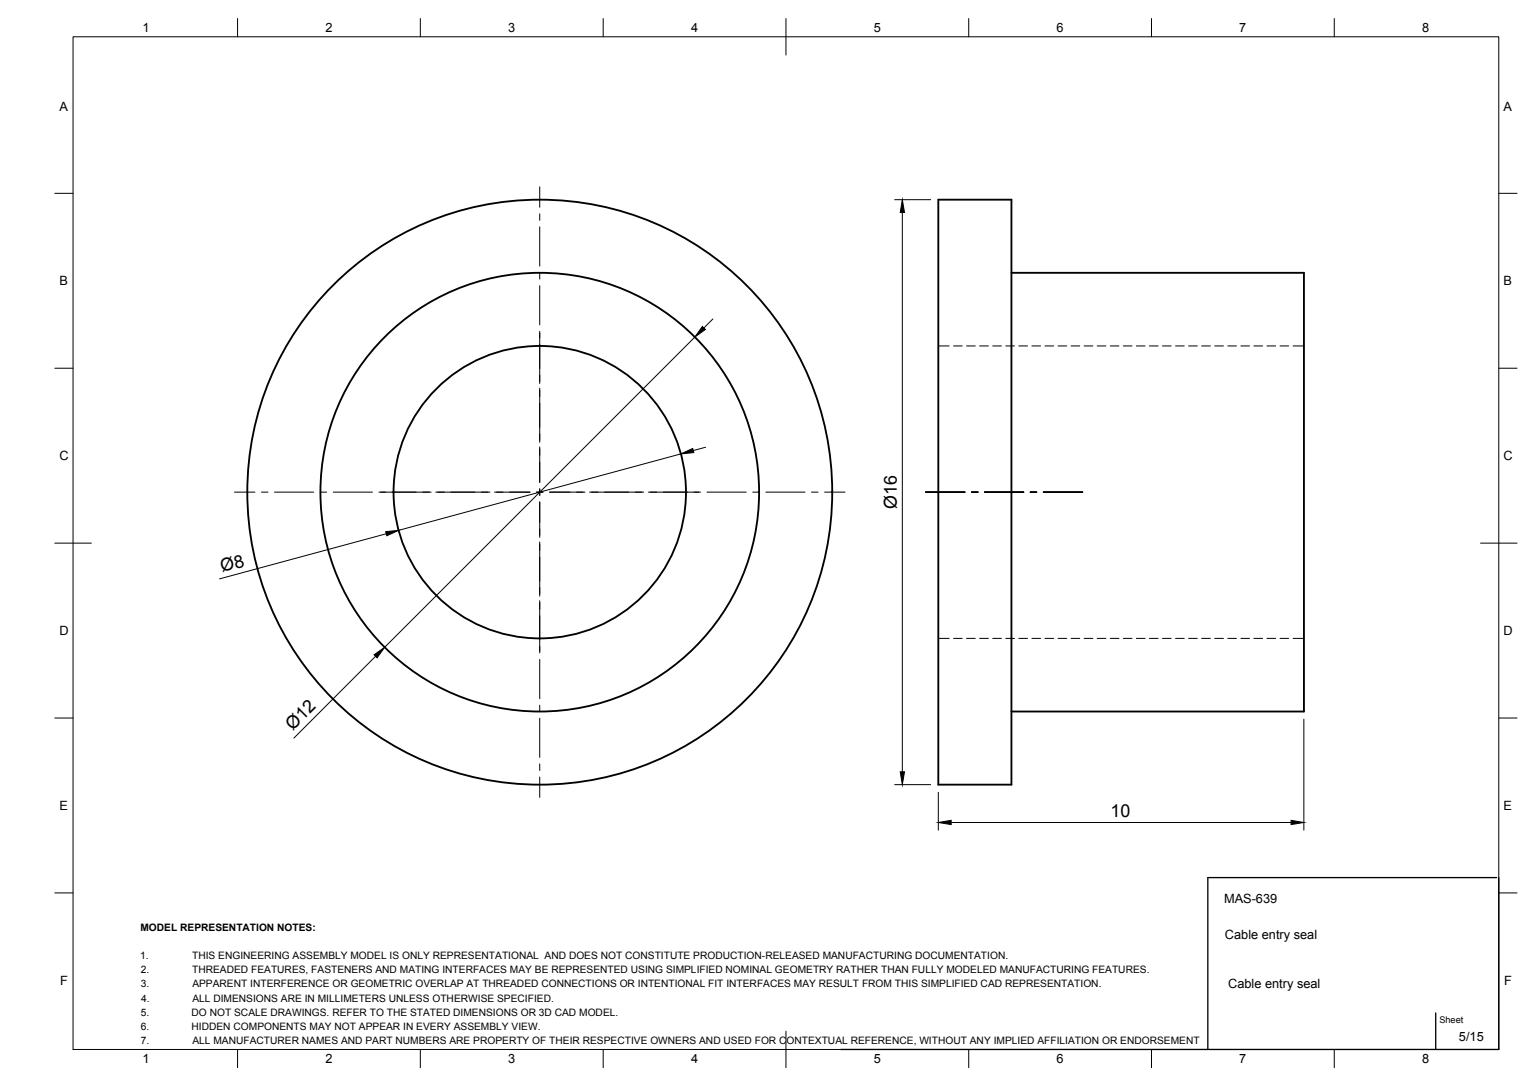
ISO-10303-21;
HEADER;
/* Generated by software containing ST-Developer
 * from STEP Tools, Inc. (www.steptools.com) 
 */

FILE_DESCRIPTION(
/* description */ ('Independent maintained push-to-latch/pull-to-reset mushroom-operator 
CAD. Two opposed spring-loaded ball detents in turned circular seats b
ias both travel stops; direct normally-closed bridge opens6mm when pre
ssed. Rounded palm/pull rim, captured head screw, removable detent clo
sures, native Coil spring families, insulated shared terminals and ord
inary machining features. Manual geometric states and ideal same-mater
ial spring-energy direction only; no electrical/safety certification, 
force/contact dynamics, wear, load or life rating. Requested blue/gray
 visual palette, not safety identification. External wiring/anchors an
d application engineering omitted.'),
/* implementation_level */ '2;1');

FILE_NAME(
/* name */ 'Cable entry seal.step',
/* time_stamp */ '2026-11-08T17:54:26-08:00',
/* author */ (''),
/* organization */ (''),
/* preprocessor_version */ 'ST-DEVELOPER v20.2',
/* originating_system */ 'Autodesk Translation Framework v15.17.0.0',
/* authorisation */ '');

FILE_SCHEMA (('AUTOMOTIVE_DESIGN { 1 0 10303 214 3 1 1 }'));
ENDSEC;

DATA;
#10=MECHANICAL_DESIGN_GEOMETRIC_PRESENTATION_REPRESENTATION('',(#192),#43980);
#158=SHAPE_REPRESENTATION_RELATIONSHIP('SRR','None',#44058,#175);
#175=ADVANCED_BREP_SHAPE_REPRESENTATION('',(#209),#43965);
#192=STYLED_ITEM('',(#44152),#209);
#209=MANIFOLD_SOLID_BREP('Body1',#11233);
#295=FACE_BOUND('',#1362,.T.);
#296=FACE_BOUND('',#1365,.T.);
#297=FACE_BOUND('',#1369,.T.);
#385=PLANE('',#11728);
#386=PLANE('',#11733);
#387=PLANE('',#11739);
#702=FACE_OUTER_BOUND('',#1361,.T.);
#703=FACE_OUTER_BOUND('',#1363,.T.);
#704=FACE_OUTER_BOUND('',#1364,.T.);
#705=FACE_OUTER_BOUND('',#1366,.T.);
#706=FACE_OUTER_BOUND('',#1367,.T.);
#707=FACE_OUTER_BOUND('',#1368,.T.);
#1361=EDGE_LOOP('',(#8063));
#1362=EDGE_LOOP('',(#8064));
#1363=EDGE_LOOP('',(#8065,#8066,#8067,#8068));
#1364=EDGE_LOOP('',(#8069));
#1365=EDGE_LOOP('',(#8070));
#1366=EDGE_LOOP('',(#8071,#8072,#8073,#8074));
#1367=EDGE_LOOP('',(#8075,#8076,#8077,#8078));
#1368=EDGE_LOOP('',(#8079));
#1369=EDGE_LOOP('',(#8080));
#1883=CIRCLE('',#11729,0.8);
#1884=CIRCLE('',#11730,0.6);
#1885=CIRCLE('',#11732,0.8);
#1886=CIRCLE('',#11734,0.4);
#1887=CIRCLE('',#11736,0.4);
#1888=CIRCLE('',#11738,0.6);
#3059=LINE('',#24801,#3691);
#3060=LINE('',#24809,#3692);
#3061=LINE('',#24813,#3693);
#3691=VECTOR('',#13088,0.8);
#3692=VECTOR('',#13099,0.4);
#3693=VECTOR('',#13104,0.6);
#4494=VERTEX_POINT('',#24795);
#4495=VERTEX_POINT('',#24797);
#4496=VERTEX_POINT('',#24800);
#4497=VERTEX_POINT('',#24804);
#4498=VERTEX_POINT('',#24807);
#4499=VERTEX_POINT('',#24811);
#5801=EDGE_CURVE('',#4494,#4494,#1883,.T.);
#5802=EDGE_CURVE('',#4495,#4495,#1884,.T.);
#5803=EDGE_CURVE('',#4494,#4496,#3059,.T.);
#5804=EDGE_CURVE('',#4496,#4496,#1885,.T.);
#5805=EDGE_CURVE('',#4497,#4497,#1886,.T.);
#5806=EDGE_CURVE('',#4498,#4498,#1887,.T.);
#5807=EDGE_CURVE('',#4498,#4497,#3060,.T.);
#5808=EDGE_CURVE('',#4499,#4499,#1888,.T.);
#5809=EDGE_CURVE('',#4499,#4495,#3061,.T.);
#8063=ORIENTED_EDGE('',*,*,#5801,.T.);
#8064=ORIENTED_EDGE('',*,*,#5802,.F.);
#8065=ORIENTED_EDGE('',*,*,#5801,.F.);
#8066=ORIENTED_EDGE('',*,*,#5803,.T.);
#8067=ORIENTED_EDGE('',*,*,#5804,.T.);
#8068=ORIENTED_EDGE('',*,*,#5803,.F.);
#8069=ORIENTED_EDGE('',*,*,#5804,.F.);
#8070=ORIENTED_EDGE('',*,*,#5805,.F.);
#8071=ORIENTED_EDGE('',*,*,#5806,.F.);
#8072=ORIENTED_EDGE('',*,*,#5807,.T.);
#8073=ORIENTED_EDGE('',*,*,#5805,.T.);
#8074=ORIENTED_EDGE('',*,*,#5807,.F.);
#8075=ORIENTED_EDGE('',*,*,#5808,.F.);
#8076=ORIENTED_EDGE('',*,*,#5809,.T.);
#8077=ORIENTED_EDGE('',*,*,#5802,.T.);
#8078=ORIENTED_EDGE('',*,*,#5809,.F.);
#8079=ORIENTED_EDGE('',*,*,#5808,.T.);
#8080=ORIENTED_EDGE('',*,*,#5806,.T.);
#10335=CYLINDRICAL_SURFACE('',#11731,0.8);
#10336=CYLINDRICAL_SURFACE('',#11735,0.4);
#10337=CYLINDRICAL_SURFACE('',#11737,0.6);
#10827=ADVANCED_FACE('',(#702,#295),#385,.T.);
#10828=ADVANCED_FACE('',(#703),#10335,.T.);
#10829=ADVANCED_FACE('',(#704,#296),#386,.F.);
#10830=ADVANCED_FACE('',(#705),#10336,.F.);
#10831=ADVANCED_FACE('',(#706),#10337,.T.);
#10832=ADVANCED_FACE('',(#707,#297),#387,.T.);
#11233=CLOSED_SHELL('',(#10827,#10828,#10829,#10830,#10831,#10832));
#11727=AXIS2_PLACEMENT_3D('',#24793,#13078,#13079);
#11728=AXIS2_PLACEMENT_3D('',#24794,#13080,#13081);
#11729=AXIS2_PLACEMENT_3D('',#24796,#13082,#13083);
#11730=AXIS2_PLACEMENT_3D('',#24798,#13084,#13085);
#11731=AXIS2_PLACEMENT_3D('',#24799,#13086,#13087);
#11732=AXIS2_PLACEMENT_3D('',#24802,#13089,#13090);
#11733=AXIS2_PLACEMENT_3D('',#24803,#13091,#13092);
#11734=AXIS2_PLACEMENT_3D('',#24805,#13093,#13094);
#11735=AXIS2_PLACEMENT_3D('',#24806,#13095,#13096);
#11736=AXIS2_PLACEMENT_3D('',#24808,#13097,#13098);
#11737=AXIS2_PLACEMENT_3D('',#24810,#13100,#13101);
#11738=AXIS2_PLACEMENT_3D('',#24812,#13102,#13103);
#11739=AXIS2_PLACEMENT_3D('',#24814,#13105,#13106);
#13078=DIRECTION('axis',(0.,0.,1.));
#13079=DIRECTION('refdir',(1.,0.,0.));
#13080=DIRECTION('center_axis',(0.,0.,1.));
#13081=DIRECTION('ref_axis',(1.,0.,0.));
#13082=DIRECTION('center_axis',(0.,0.,1.));
#13083=DIRECTION('ref_axis',(1.,0.,0.));
#13084=DIRECTION('center_axis',(0.,0.,1.));
#13085=DIRECTION('ref_axis',(1.,0.,0.));
#13086=DIRECTION('center_axis',(0.,0.,1.));
#13087=DIRECTION('ref_axis',(1.,0.,0.));
#13088=DIRECTION('',(0.,0.,-1.));
#13089=DIRECTION('center_axis',(0.,0.,1.));
#13090=DIRECTION('ref_axis',(1.,0.,0.));
#13091=DIRECTION('center_axis',(0.,0.,1.));
#13092=DIRECTION('ref_axis',(1.,0.,0.));
#13093=DIRECTION('center_axis',(0.,0.,-1.));
#13094=DIRECTION('ref_axis',(1.,0.,0.));
#13095=DIRECTION('center_axis',(0.,0.,1.));
#13096=DIRECTION('ref_axis',(1.,0.,0.));
#13097=DIRECTION('center_axis',(0.,0.,-1.));
#13098=DIRECTION('ref_axis',(1.,0.,0.));
#13099=DIRECTION('',(0.,0.,-1.));
#13100=DIRECTION('center_axis',(0.,0.,1.));
#13101=DIRECTION('ref_axis',(1.,0.,0.));
#13102=DIRECTION('center_axis',(0.,0.,1.));
#13103=DIRECTION('ref_axis',(1.,0.,0.));
#13104=DIRECTION('',(0.,0.,-1.));
#13105=DIRECTION('center_axis',(0.,0.,1.));
#13106=DIRECTION('ref_axis',(1.,0.,0.));
#24793=CARTESIAN_POINT('',(0.,0.,0.));
#24794=CARTESIAN_POINT('Origin',(0.,0.,0.));
#24795=CARTESIAN_POINT('',(-0.8,-9.79717439317883E-17,0.));
#24796=CARTESIAN_POINT('Origin',(0.,0.,0.));
#24797=CARTESIAN_POINT('',(-0.6,-7.34788079488412E-17,0.));
#24798=CARTESIAN_POINT('Origin',(0.,0.,0.));
#24799=CARTESIAN_POINT('Origin',(0.,0.,-0.2));
#24800=CARTESIAN_POINT('',(-0.8,-9.79717439317883E-17,-0.2));
#24801=CARTESIAN_POINT('',(-0.8,-9.79717439317883E-17,-0.2));
#24802=CARTESIAN_POINT('Origin',(0.,0.,-0.2));
#24803=CARTESIAN_POINT('Origin',(0.,0.,-0.2));
#24804=CARTESIAN_POINT('',(-0.4,-4.89858719658941E-17,-0.2));
#24805=CARTESIAN_POINT('Origin',(0.,0.,-0.2));
#24806=CARTESIAN_POINT('Origin',(0.,0.,0.));
#24807=CARTESIAN_POINT('',(-0.4,-4.89858719658941E-17,0.8));
#24808=CARTESIAN_POINT('Origin',(0.,0.,0.8));
#24809=CARTESIAN_POINT('',(-0.4,-4.89858719658941E-17,0.));
#24810=CARTESIAN_POINT('Origin',(0.,0.,0.));
#24811=CARTESIAN_POINT('',(-0.6,-7.34788079488412E-17,0.8));
#24812=CARTESIAN_POINT('Origin',(0.,0.,0.8));
#24813=CARTESIAN_POINT('',(-0.6,-7.34788079488412E-17,0.));
#24814=CARTESIAN_POINT('Origin',(0.,0.,0.8));
#43946=UNCERTAINTY_MEASURE_WITH_UNIT(LENGTH_MEASURE(0.001),#43981,
'DISTANCE_ACCURACY_VALUE',
'Maximum model space distance between geometric entities at asserted c
onnectivities');
#43961=UNCERTAINTY_MEASURE_WITH_UNIT(LENGTH_MEASURE(0.001),#43981,
'DISTANCE_ACCURACY_VALUE',
'Maximum model space distance between geometric entities at asserted c
onnectivities');
#43965=(
GEOMETRIC_REPRESENTATION_CONTEXT(3)
GLOBAL_UNCERTAINTY_ASSIGNED_CONTEXT((#43946))
GLOBAL_UNIT_ASSIGNED_CONTEXT((#43981,#43983,#43984))
REPRESENTATION_CONTEXT('','3D')
);
#43980=(
GEOMETRIC_REPRESENTATION_CONTEXT(3)
GLOBAL_UNCERTAINTY_ASSIGNED_CONTEXT((#43961))
GLOBAL_UNIT_ASSIGNED_CONTEXT((#43981,#43983,#43984))
REPRESENTATION_CONTEXT('','3D')
);
#43981=(
LENGTH_UNIT()
NAMED_UNIT(*)
SI_UNIT(.CENTI.,.METRE.)
);
#43983=(
NAMED_UNIT(*)
PLANE_ANGLE_UNIT()
SI_UNIT($,.RADIAN.)
);
#43984=(
NAMED_UNIT(*)
SI_UNIT($,.STERADIAN.)
SOLID_ANGLE_UNIT()
);
#43988=SHAPE_DEFINITION_REPRESENTATION(#44006,#44058);
#44006=PRODUCT_DEFINITION_SHAPE('',$,#44077);
#44058=SHAPE_REPRESENTATION('',(#11727),#43965);
#44073=PRODUCT_DEFINITION_CONTEXT('part definition',#44129,'design');
#44077=PRODUCT_DEFINITION('Cable entry seal','Cable entry seal',#44095,
#44073);
#44095=PRODUCT_DEFINITION_FORMATION('',$,#44134);
#44129=APPLICATION_CONTEXT(
'Core Data for Automotive Mechanical Design Process');
#44130=PRODUCT_CONTEXT('part definition',#44129,'mechanical');
#44134=PRODUCT('Cable entry seal','Cable entry seal',$,(#44130));
#44152=PRESENTATION_STYLE_ASSIGNMENT((#44164));
#44164=SURFACE_STYLE_USAGE(.BOTH.,#44176);
#44176=SURFACE_SIDE_STYLE('',(#44188));
#44188=SURFACE_STYLE_FILL_AREA(#44200);
#44200=FILL_AREA_STYLE('Charcoal',(#44212));
#44212=FILL_AREA_STYLE_COLOUR('Charcoal',#44224);
#44224=COLOUR_RGB('Charcoal',0.164705882352941,0.184313725490196,0.211764705882353);
ENDSEC;
END-ISO-10303-21;
